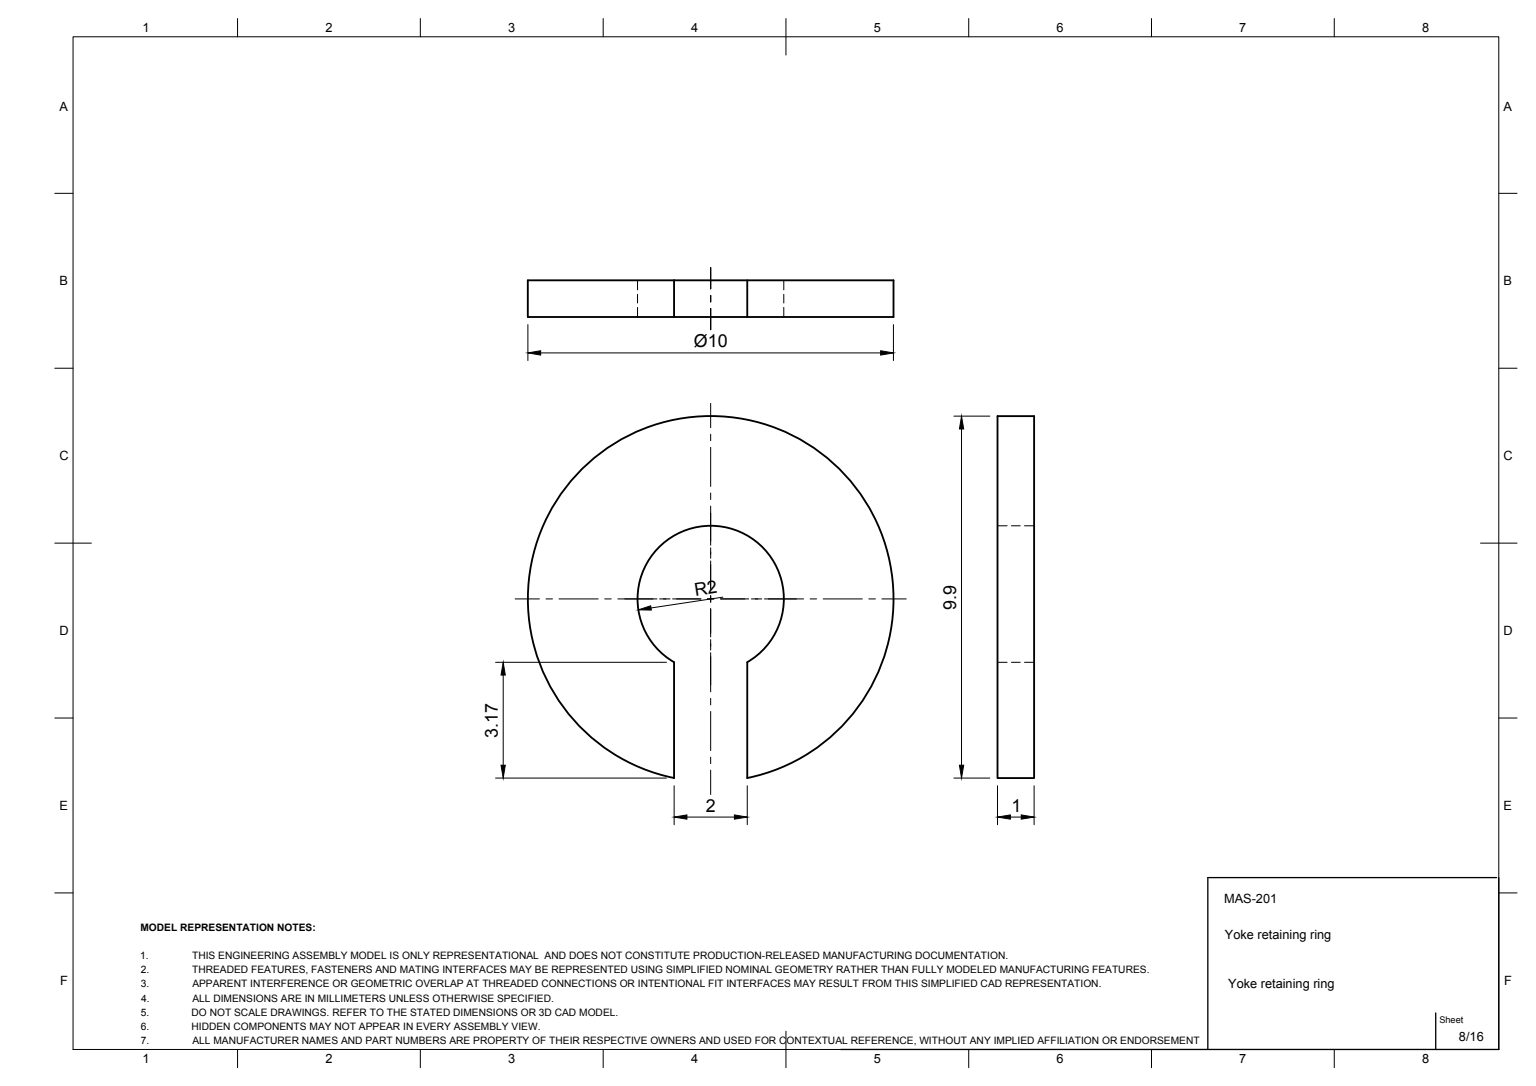
ISO-10303-21;
HEADER;
/* Generated by software containing ST-Developer
 * from STEP Tools, Inc. (www.steptools.com) 
 */

FILE_DESCRIPTION(
/* description */ ('Independent manual two-gate roller-track escapement for nominal30mm d
iameter20mm wide feed rollers. Opposed gates are driven by native capt
ured pin-slot loops with positive curved-slot travel stops at\X\B116de
g. Repeated gate/pin/washer/clip instances, adapted native common bear
ing families, full retaining lips and rotating polymer grip. External 
workpieces, gravity feeder/incline and mount anchors outside assembly.
 No powered-feed compatibility, impact, capacity, safety, force, wear 
or life rating.'),
/* implementation_level */ '2;1');

FILE_NAME(
/* name */ 'Yoke retaining ring.step',
/* time_stamp */ '2026-11-08T18:43:23-08:00',
/* author */ (''),
/* organization */ (''),
/* preprocessor_version */ 'ST-DEVELOPER v20.2',
/* originating_system */ 'Autodesk Translation Framework v15.17.0.0',
/* authorisation */ '');

FILE_SCHEMA (('AUTOMOTIVE_DESIGN { 1 0 10303 214 3 1 1 }'));
ENDSEC;

DATA;
#10=MECHANICAL_DESIGN_GEOMETRIC_PRESENTATION_REPRESENTATION('',(#462),#19863);
#424=SHAPE_REPRESENTATION_RELATIONSHIP('SRR','None',#19942,#443);
#443=ADVANCED_BREP_SHAPE_REPRESENTATION('',(#481),#19851);
#462=STYLED_ITEM('',(#20044),#481);
#481=MANIFOLD_SOLID_BREP('Body1',#6431);
#836=LINE('',#15847,#1301);
#837=LINE('',#15849,#1302);
#838=LINE('',#15851,#1303);
#839=LINE('',#15852,#1304);
#840=LINE('',#15856,#1305);
#841=LINE('',#15858,#1306);
#842=LINE('',#15860,#1307);
#843=LINE('',#15861,#1308);
#1301=VECTOR('',#8174,10.);
#1302=VECTOR('',#8175,10.);
#1303=VECTOR('',#8176,10.);
#1304=VECTOR('',#8177,10.);
#1305=VECTOR('',#8180,10.);
#1306=VECTOR('',#8181,10.);
#1307=VECTOR('',#8182,10.);
#1308=VECTOR('',#8183,10.);
#1546=CYLINDRICAL_SURFACE('',#6977,2.);
#1547=CYLINDRICAL_SURFACE('',#6979,5.);
#1919=FACE_OUTER_BOUND('',#2328,.T.);
#1920=FACE_OUTER_BOUND('',#2329,.T.);
#1921=FACE_OUTER_BOUND('',#2330,.T.);
#1922=FACE_OUTER_BOUND('',#2331,.T.);
#1923=FACE_OUTER_BOUND('',#2332,.T.);
#1924=FACE_OUTER_BOUND('',#2333,.T.);
#2328=EDGE_LOOP('',(#5349,#5350,#5351,#5352));
#2329=EDGE_LOOP('',(#5353,#5354,#5355,#5356));
#2330=EDGE_LOOP('',(#5357,#5358,#5359,#5360));
#2331=EDGE_LOOP('',(#5361,#5362,#5363,#5364));
#2332=EDGE_LOOP('',(#5365,#5366,#5367,#5368));
#2333=EDGE_LOOP('',(#5369,#5370,#5371,#5372));
#2558=CIRCLE('',#6975,5.);
#2559=CIRCLE('',#6976,2.);
#2560=CIRCLE('',#6978,2.);
#2561=CIRCLE('',#6980,5.);
#3028=VERTEX_POINT('',#15845);
#3029=VERTEX_POINT('',#15846);
#3030=VERTEX_POINT('',#15848);
#3031=VERTEX_POINT('',#15850);
#3032=VERTEX_POINT('',#15854);
#3033=VERTEX_POINT('',#15855);
#3034=VERTEX_POINT('',#15857);
#3035=VERTEX_POINT('',#15859);
#3833=EDGE_CURVE('',#3028,#3029,#836,.T.);
#3834=EDGE_CURVE('',#3030,#3028,#837,.T.);
#3835=EDGE_CURVE('',#3031,#3030,#838,.T.);
#3836=EDGE_CURVE('',#3029,#3031,#839,.T.);
#3837=EDGE_CURVE('',#3032,#3033,#840,.T.);
#3838=EDGE_CURVE('',#3034,#3032,#841,.T.);
#3839=EDGE_CURVE('',#3035,#3034,#842,.T.);
#3840=EDGE_CURVE('',#3033,#3035,#843,.T.);
#3841=EDGE_CURVE('',#3030,#3035,#2558,.T.);
#3842=EDGE_CURVE('',#3033,#3028,#2559,.T.);
#3843=EDGE_CURVE('',#3032,#3029,#2560,.T.);
#3844=EDGE_CURVE('',#3031,#3034,#2561,.T.);
#5349=ORIENTED_EDGE('',*,*,#3833,.F.);
#5350=ORIENTED_EDGE('',*,*,#3834,.F.);
#5351=ORIENTED_EDGE('',*,*,#3835,.F.);
#5352=ORIENTED_EDGE('',*,*,#3836,.F.);
#5353=ORIENTED_EDGE('',*,*,#3837,.F.);
#5354=ORIENTED_EDGE('',*,*,#3838,.F.);
#5355=ORIENTED_EDGE('',*,*,#3839,.F.);
#5356=ORIENTED_EDGE('',*,*,#3840,.F.);
#5357=ORIENTED_EDGE('',*,*,#3840,.T.);
#5358=ORIENTED_EDGE('',*,*,#3841,.F.);
#5359=ORIENTED_EDGE('',*,*,#3834,.T.);
#5360=ORIENTED_EDGE('',*,*,#3842,.F.);
#5361=ORIENTED_EDGE('',*,*,#3837,.T.);
#5362=ORIENTED_EDGE('',*,*,#3842,.T.);
#5363=ORIENTED_EDGE('',*,*,#3833,.T.);
#5364=ORIENTED_EDGE('',*,*,#3843,.F.);
#5365=ORIENTED_EDGE('',*,*,#3839,.T.);
#5366=ORIENTED_EDGE('',*,*,#3844,.F.);
#5367=ORIENTED_EDGE('',*,*,#3835,.T.);
#5368=ORIENTED_EDGE('',*,*,#3841,.T.);
#5369=ORIENTED_EDGE('',*,*,#3838,.T.);
#5370=ORIENTED_EDGE('',*,*,#3843,.T.);
#5371=ORIENTED_EDGE('',*,*,#3836,.T.);
#5372=ORIENTED_EDGE('',*,*,#3844,.T.);
#6016=PLANE('',#6972);
#6017=PLANE('',#6973);
#6018=PLANE('',#6974);
#6019=PLANE('',#6981);
#6298=ADVANCED_FACE('',(#1919),#6016,.F.);
#6299=ADVANCED_FACE('',(#1920),#6017,.F.);
#6300=ADVANCED_FACE('',(#1921),#6018,.F.);
#6301=ADVANCED_FACE('',(#1922),#1546,.F.);
#6302=ADVANCED_FACE('',(#1923),#1547,.T.);
#6303=ADVANCED_FACE('',(#1924),#6019,.T.);
#6431=CLOSED_SHELL('',(#6298,#6299,#6300,#6301,#6302,#6303));
#6971=AXIS2_PLACEMENT_3D('',#15843,#8170,#8171);
#6972=AXIS2_PLACEMENT_3D('',#15844,#8172,#8173);
#6973=AXIS2_PLACEMENT_3D('',#15853,#8178,#8179);
#6974=AXIS2_PLACEMENT_3D('',#15862,#8184,#8185);
#6975=AXIS2_PLACEMENT_3D('',#15863,#8186,#8187);
#6976=AXIS2_PLACEMENT_3D('',#15864,#8188,#8189);
#6977=AXIS2_PLACEMENT_3D('',#15865,#8190,#8191);
#6978=AXIS2_PLACEMENT_3D('',#15866,#8192,#8193);
#6979=AXIS2_PLACEMENT_3D('',#15867,#8194,#8195);
#6980=AXIS2_PLACEMENT_3D('',#15868,#8196,#8197);
#6981=AXIS2_PLACEMENT_3D('',#15869,#8198,#8199);
#8170=DIRECTION('axis',(0.,0.,1.));
#8171=DIRECTION('refdir',(1.,0.,0.));
#8172=DIRECTION('center_axis',(-1.,0.,0.));
#8173=DIRECTION('ref_axis',(0.,1.,0.));
#8174=DIRECTION('',(0.,0.,1.));
#8175=DIRECTION('',(0.,-1.,0.));
#8176=DIRECTION('',(0.,0.,-1.));
#8177=DIRECTION('',(0.,1.,0.));
#8178=DIRECTION('center_axis',(1.,0.,0.));
#8179=DIRECTION('ref_axis',(0.,-1.,0.));
#8180=DIRECTION('',(0.,0.,-1.));
#8181=DIRECTION('',(0.,-1.,0.));
#8182=DIRECTION('',(0.,0.,1.));
#8183=DIRECTION('',(0.,1.,0.));
#8184=DIRECTION('center_axis',(0.,0.,1.));
#8185=DIRECTION('ref_axis',(1.,0.,0.));
#8186=DIRECTION('center_axis',(0.,0.,1.));
#8187=DIRECTION('ref_axis',(1.,0.,0.));
#8188=DIRECTION('center_axis',(0.,0.,-1.));
#8189=DIRECTION('ref_axis',(1.,0.,0.));
#8190=DIRECTION('center_axis',(0.,0.,1.));
#8191=DIRECTION('ref_axis',(6.12323399573677E-17,-1.,0.));
#8192=DIRECTION('center_axis',(0.,0.,-1.));
#8193=DIRECTION('ref_axis',(1.,0.,0.));
#8194=DIRECTION('center_axis',(0.,0.,1.));
#8195=DIRECTION('ref_axis',(6.12323399573677E-17,-1.,0.));
#8196=DIRECTION('center_axis',(0.,0.,1.));
#8197=DIRECTION('ref_axis',(1.,0.,0.));
#8198=DIRECTION('center_axis',(0.,0.,1.));
#8199=DIRECTION('ref_axis',(1.,0.,0.));
#15843=CARTESIAN_POINT('',(0.,0.,0.));
#15844=CARTESIAN_POINT('Origin',(-1.,0.,1.));
#15845=CARTESIAN_POINT('',(-1.,1.73205080756888,0.));
#15846=CARTESIAN_POINT('',(-1.,1.73205080756888,1.));
#15847=CARTESIAN_POINT('',(-1.,1.73205080756888,0.));
#15848=CARTESIAN_POINT('',(-1.,4.89897948556636,0.));
#15849=CARTESIAN_POINT('',(-1.,0.,0.));
#15850=CARTESIAN_POINT('',(-1.,4.89897948556636,1.));
#15851=CARTESIAN_POINT('',(-1.,4.89897948556636,0.));
#15852=CARTESIAN_POINT('',(-1.,0.,1.));
#15853=CARTESIAN_POINT('Origin',(1.,10.,1.));
#15854=CARTESIAN_POINT('',(1.,1.73205080756888,1.));
#15855=CARTESIAN_POINT('',(1.,1.73205080756888,0.));
#15856=CARTESIAN_POINT('',(1.,1.73205080756888,0.));
#15857=CARTESIAN_POINT('',(1.,4.89897948556636,1.));
#15858=CARTESIAN_POINT('',(1.,5.,1.));
#15859=CARTESIAN_POINT('',(1.,4.89897948556636,0.));
#15860=CARTESIAN_POINT('',(1.,4.89897948556636,0.));
#15861=CARTESIAN_POINT('',(1.,5.,0.));
#15862=CARTESIAN_POINT('Origin',(0.,0.,0.));
#15863=CARTESIAN_POINT('Origin',(0.,0.,0.));
#15864=CARTESIAN_POINT('Origin',(0.,0.,0.));
#15865=CARTESIAN_POINT('Origin',(0.,0.,0.));
#15866=CARTESIAN_POINT('Origin',(0.,0.,1.));
#15867=CARTESIAN_POINT('Origin',(0.,0.,0.));
#15868=CARTESIAN_POINT('Origin',(0.,0.,1.));
#15869=CARTESIAN_POINT('Origin',(0.,0.,1.));
#19830=UNCERTAINTY_MEASURE_WITH_UNIT(LENGTH_MEASURE(0.01),#19864,
'DISTANCE_ACCURACY_VALUE',
'Maximum model space distance between geometric entities at asserted c
onnectivities');
#19842=UNCERTAINTY_MEASURE_WITH_UNIT(LENGTH_MEASURE(0.01),#19864,
'DISTANCE_ACCURACY_VALUE',
'Maximum model space distance between geometric entities at asserted c
onnectivities');
#19851=(
GEOMETRIC_REPRESENTATION_CONTEXT(3)
GLOBAL_UNCERTAINTY_ASSIGNED_CONTEXT((#19830))
GLOBAL_UNIT_ASSIGNED_CONTEXT((#19864,#19866,#19867))
REPRESENTATION_CONTEXT('','3D')
);
#19863=(
GEOMETRIC_REPRESENTATION_CONTEXT(3)
GLOBAL_UNCERTAINTY_ASSIGNED_CONTEXT((#19842))
GLOBAL_UNIT_ASSIGNED_CONTEXT((#19864,#19866,#19867))
REPRESENTATION_CONTEXT('','3D')
);
#19864=(
LENGTH_UNIT()
NAMED_UNIT(*)
SI_UNIT(.MILLI.,.METRE.)
);
#19866=(
NAMED_UNIT(*)
PLANE_ANGLE_UNIT()
SI_UNIT($,.RADIAN.)
);
#19867=(
NAMED_UNIT(*)
SI_UNIT($,.STERADIAN.)
SOLID_ANGLE_UNIT()
);
#19876=SHAPE_DEFINITION_REPRESENTATION(#19896,#19942);
#19896=PRODUCT_DEFINITION_SHAPE('',$,#19963);
#19942=SHAPE_REPRESENTATION('',(#6971),#19851);
#19954=PRODUCT_DEFINITION_CONTEXT('part definition',#20016,'design');
#19963=PRODUCT_DEFINITION('Yoke retaining ring','Yoke retaining ring',#19983,
#19954);
#19983=PRODUCT_DEFINITION_FORMATION('',$,#20026);
#20016=APPLICATION_CONTEXT(
'Core Data for Automotive Mechanical Design Process');
#20017=PRODUCT_CONTEXT('part definition',#20016,'mechanical');
#20026=PRODUCT('Yoke retaining ring','Yoke retaining ring',$,(#20017));
#20044=PRESENTATION_STYLE_ASSIGNMENT((#20051));
#20051=SURFACE_STYLE_USAGE(.BOTH.,#20058);
#20058=SURFACE_SIDE_STYLE('',(#20065));
#20065=SURFACE_STYLE_FILL_AREA(#20072);
#20072=FILL_AREA_STYLE('Dark gray',(#20079));
#20079=FILL_AREA_STYLE_COLOUR('Dark gray',#20086);
#20086=COLOUR_RGB('Dark gray',0.250980392156863,0.282352941176471,0.32156862745098);
ENDSEC;
END-ISO-10303-21;
